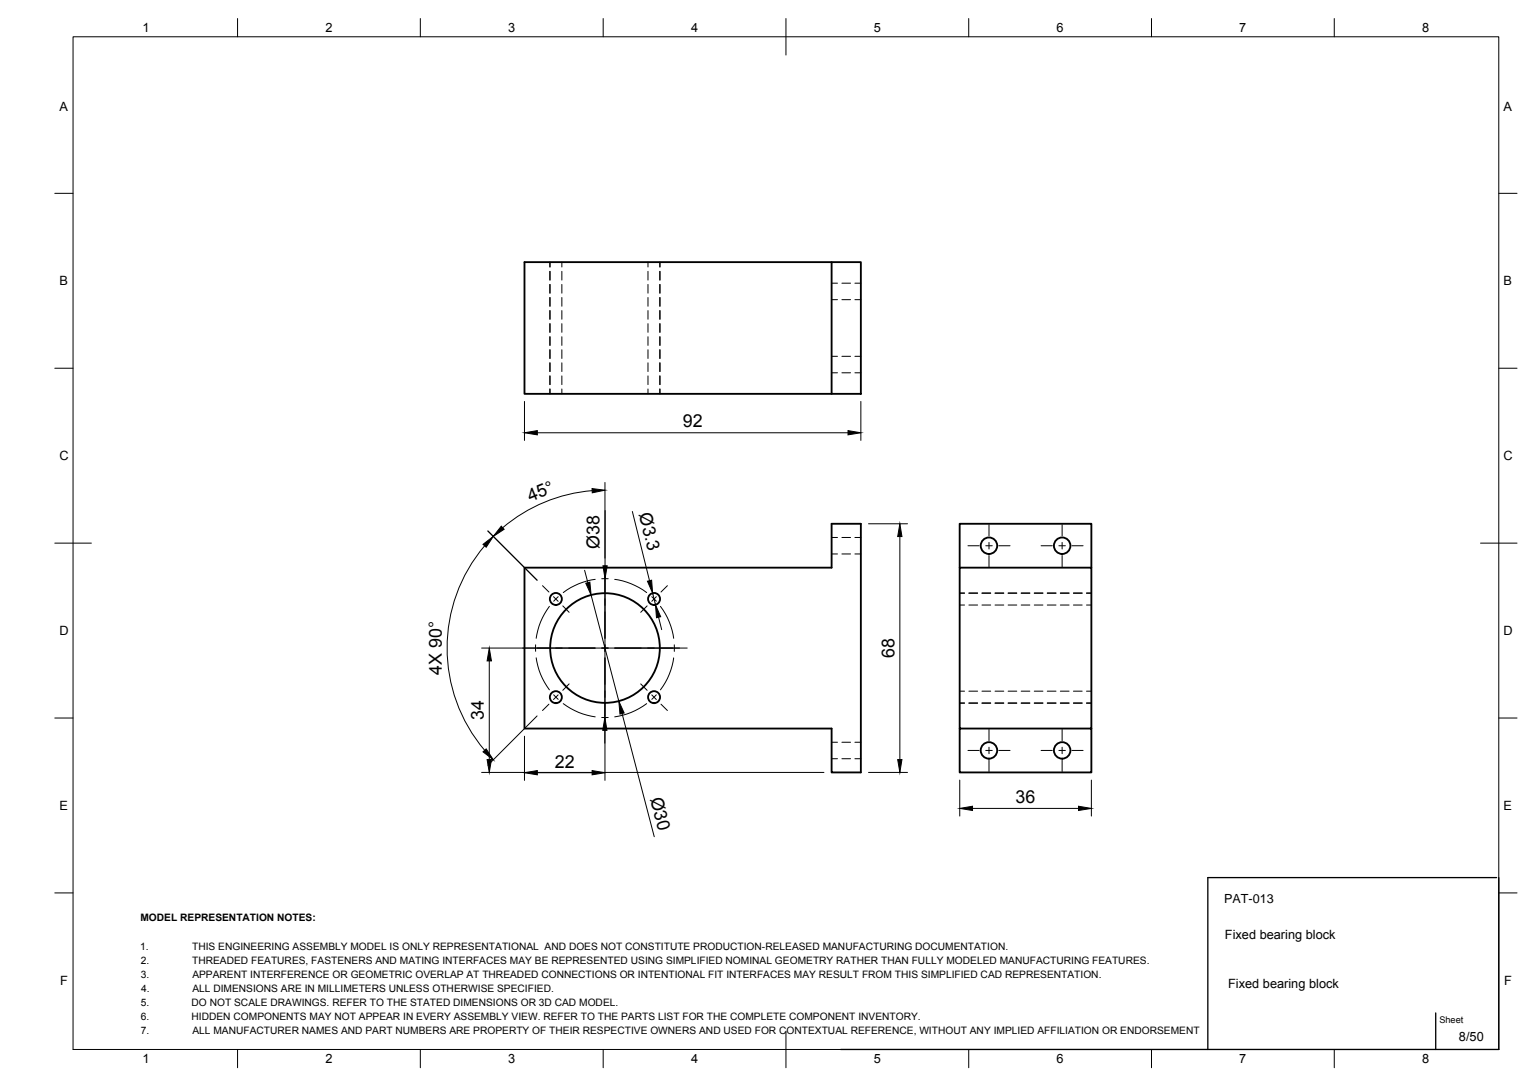
ISO-10303-21;
HEADER;
/* Generated by software containing ST-Developer
 * from STEP Tools, Inc. (www.steptools.com) 
 */

FILE_DESCRIPTION(
/* description */ ('Belt-driven linear axis on 2020 extrusion'),
/* implementation_level */ '2;1');

FILE_NAME(
/* name */ 'Fixed bearing block.step',
/* time_stamp */ '2026-10-28T03:26:09-07:00',
/* author */ (''),
/* organization */ (''),
/* preprocessor_version */ 'ST-DEVELOPER v20.2',
/* originating_system */ 'Autodesk Translation Framework v15.17.0.0',
/* authorisation */ '');

FILE_SCHEMA (('AUTOMOTIVE_DESIGN { 1 0 10303 214 3 1 1 }'));
ENDSEC;

DATA;
#10=MECHANICAL_DESIGN_GEOMETRIC_PRESENTATION_REPRESENTATION('',(#615),#20096);
#521=SHAPE_REPRESENTATION_RELATIONSHIP('SRR','None',#20317,#567);
#567=ADVANCED_BREP_SHAPE_REPRESENTATION('',(#671),#20048);
#615=STYLED_ITEM('',(#20650),#671);
#671=MANIFOLD_SOLID_BREP('Body1',#10928);
#742=FACE_BOUND('',#1972,.T.);
#743=FACE_BOUND('',#1973,.T.);
#744=FACE_BOUND('',#1975,.T.);
#745=FACE_BOUND('',#1976,.T.);
#746=FACE_BOUND('',#1980,.T.);
#747=FACE_BOUND('',#1981,.T.);
#748=FACE_BOUND('',#1982,.T.);
#749=FACE_BOUND('',#1983,.T.);
#750=FACE_BOUND('',#1984,.T.);
#751=FACE_BOUND('',#1987,.T.);
#752=FACE_BOUND('',#1988,.T.);
#753=FACE_BOUND('',#1989,.T.);
#754=FACE_BOUND('',#1990,.T.);
#755=FACE_BOUND('',#1991,.T.);
#756=FACE_BOUND('',#1995,.T.);
#757=FACE_BOUND('',#1996,.T.);
#758=FACE_BOUND('',#1997,.T.);
#759=FACE_BOUND('',#1998,.T.);
#935=PLANE('',#11629);
#936=PLANE('',#11630);
#937=PLANE('',#11631);
#938=PLANE('',#11632);
#939=PLANE('',#11633);
#940=PLANE('',#11634);
#941=PLANE('',#11635);
#942=PLANE('',#11636);
#943=PLANE('',#11637);
#944=PLANE('',#11638);
#1316=FACE_OUTER_BOUND('',#1962,.T.);
#1317=FACE_OUTER_BOUND('',#1963,.T.);
#1318=FACE_OUTER_BOUND('',#1964,.T.);
#1319=FACE_OUTER_BOUND('',#1965,.T.);
#1320=FACE_OUTER_BOUND('',#1966,.T.);
#1321=FACE_OUTER_BOUND('',#1967,.T.);
#1322=FACE_OUTER_BOUND('',#1968,.T.);
#1323=FACE_OUTER_BOUND('',#1969,.T.);
#1324=FACE_OUTER_BOUND('',#1970,.T.);
#1325=FACE_OUTER_BOUND('',#1971,.T.);
#1326=FACE_OUTER_BOUND('',#1974,.T.);
#1327=FACE_OUTER_BOUND('',#1977,.T.);
#1328=FACE_OUTER_BOUND('',#1978,.T.);
#1329=FACE_OUTER_BOUND('',#1979,.T.);
#1330=FACE_OUTER_BOUND('',#1985,.T.);
#1331=FACE_OUTER_BOUND('',#1986,.T.);
#1332=FACE_OUTER_BOUND('',#1992,.T.);
#1333=FACE_OUTER_BOUND('',#1993,.T.);
#1334=FACE_OUTER_BOUND('',#1994,.T.);
#1962=EDGE_LOOP('',(#7493,#7494,#7495,#7496));
#1963=EDGE_LOOP('',(#7497,#7498,#7499,#7500));
#1964=EDGE_LOOP('',(#7501,#7502,#7503,#7504));
#1965=EDGE_LOOP('',(#7505,#7506,#7507,#7508));
#1966=EDGE_LOOP('',(#7509,#7510,#7511,#7512));
#1967=EDGE_LOOP('',(#7513,#7514,#7515,#7516));
#1968=EDGE_LOOP('',(#7517,#7518,#7519,#7520));
#1969=EDGE_LOOP('',(#7521,#7522,#7523,#7524));
#1970=EDGE_LOOP('',(#7525,#7526,#7527,#7528));
#1971=EDGE_LOOP('',(#7529,#7530,#7531,#7532));
#1972=EDGE_LOOP('',(#7533));
#1973=EDGE_LOOP('',(#7534));
#1974=EDGE_LOOP('',(#7535,#7536,#7537,#7538));
#1975=EDGE_LOOP('',(#7539));
#1976=EDGE_LOOP('',(#7540));
#1977=EDGE_LOOP('',(#7541,#7542,#7543,#7544));
#1978=EDGE_LOOP('',(#7545,#7546,#7547,#7548));
#1979=EDGE_LOOP('',(#7549,#7550,#7551,#7552,#7553,#7554,#7555,#7556));
#1980=EDGE_LOOP('',(#7557));
#1981=EDGE_LOOP('',(#7558));
#1982=EDGE_LOOP('',(#7559));
#1983=EDGE_LOOP('',(#7560));
#1984=EDGE_LOOP('',(#7561));
#1985=EDGE_LOOP('',(#7562,#7563,#7564,#7565));
#1986=EDGE_LOOP('',(#7566,#7567,#7568,#7569,#7570,#7571,#7572,#7573));
#1987=EDGE_LOOP('',(#7574));
#1988=EDGE_LOOP('',(#7575));
#1989=EDGE_LOOP('',(#7576));
#1990=EDGE_LOOP('',(#7577));
#1991=EDGE_LOOP('',(#7578));
#1992=EDGE_LOOP('',(#7579,#7580,#7581,#7582));
#1993=EDGE_LOOP('',(#7583,#7584,#7585,#7586));
#1994=EDGE_LOOP('',(#7587,#7588,#7589,#7590));
#1995=EDGE_LOOP('',(#7591));
#1996=EDGE_LOOP('',(#7592));
#1997=EDGE_LOOP('',(#7593));
#1998=EDGE_LOOP('',(#7594));
#2745=LINE('',#16508,#3602);
#2746=LINE('',#16514,#3603);
#2747=LINE('',#16520,#3604);
#2748=LINE('',#16526,#3605);
#2749=LINE('',#16532,#3606);
#2750=LINE('',#16538,#3607);
#2751=LINE('',#16544,#3608);
#2752=LINE('',#16550,#3609);
#2753=LINE('',#16556,#3610);
#2754=LINE('',#16561,#3611);
#2755=LINE('',#16563,#3612);
#2756=LINE('',#16565,#3613);
#2757=LINE('',#16566,#3614);
#2758=LINE('',#16570,#3615);
#2759=LINE('',#16572,#3616);
#2760=LINE('',#16574,#3617);
#2761=LINE('',#16575,#3618);
#2762=LINE('',#16578,#3619);
#2763=LINE('',#16580,#3620);
#2764=LINE('',#16581,#3621);
#2765=LINE('',#16584,#3622);
#2766=LINE('',#16586,#3623);
#2767=LINE('',#16587,#3624);
#2768=LINE('',#16590,#3625);
#2769=LINE('',#16592,#3626);
#2770=LINE('',#16593,#3627);
#2771=LINE('',#16594,#3628);
#2772=LINE('',#16597,#3629);
#2773=LINE('',#16598,#3630);
#2774=LINE('',#16601,#3631);
#2775=LINE('',#16602,#3632);
#2776=LINE('',#16603,#3633);
#2777=LINE('',#16605,#3634);
#3602=VECTOR('',#13093,0.165);
#3603=VECTOR('',#13100,0.165);
#3604=VECTOR('',#13107,0.165);
#3605=VECTOR('',#13114,0.165);
#3606=VECTOR('',#13121,1.5);
#3607=VECTOR('',#13128,0.225);
#3608=VECTOR('',#13135,0.225);
#3609=VECTOR('',#13142,0.225);
#3610=VECTOR('',#13149,0.225);
#3611=VECTOR('',#13154,1.);
#3612=VECTOR('',#13155,1.);
#3613=VECTOR('',#13156,1.);
#3614=VECTOR('',#13157,1.);
#3615=VECTOR('',#13160,1.);
#3616=VECTOR('',#13161,1.);
#3617=VECTOR('',#13162,1.);
#3618=VECTOR('',#13163,1.);
#3619=VECTOR('',#13166,1.);
#3620=VECTOR('',#13167,1.);
#3621=VECTOR('',#13168,1.);
#3622=VECTOR('',#13171,1.);
#3623=VECTOR('',#13172,1.);
#3624=VECTOR('',#13173,1.);
#3625=VECTOR('',#13176,1.);
#3626=VECTOR('',#13177,1.);
#3627=VECTOR('',#13178,1.);
#3628=VECTOR('',#13179,1.);
#3629=VECTOR('',#13182,1.);
#3630=VECTOR('',#13183,1.);
#3631=VECTOR('',#13186,1.);
#3632=VECTOR('',#13187,1.);
#3633=VECTOR('',#13188,1.);
#3634=VECTOR('',#13191,1.);
#4419=CIRCLE('',#11603,0.165);
#4420=CIRCLE('',#11604,0.165);
#4421=CIRCLE('',#11606,0.165);
#4422=CIRCLE('',#11607,0.165);
#4423=CIRCLE('',#11609,0.165);
#4424=CIRCLE('',#11610,0.165);
#4425=CIRCLE('',#11612,0.165);
#4426=CIRCLE('',#11613,0.165);
#4427=CIRCLE('',#11615,1.5);
#4428=CIRCLE('',#11616,1.5);
#4429=CIRCLE('',#11618,0.225);
#4430=CIRCLE('',#11619,0.225);
#4431=CIRCLE('',#11621,0.225);
#4432=CIRCLE('',#11622,0.225);
#4433=CIRCLE('',#11624,0.225);
#4434=CIRCLE('',#11625,0.225);
#4435=CIRCLE('',#11627,0.225);
#4436=CIRCLE('',#11628,0.225);
#4972=VERTEX_POINT('',#16505);
#4973=VERTEX_POINT('',#16507);
#4974=VERTEX_POINT('',#16511);
#4975=VERTEX_POINT('',#16513);
#4976=VERTEX_POINT('',#16517);
#4977=VERTEX_POINT('',#16519);
#4978=VERTEX_POINT('',#16523);
#4979=VERTEX_POINT('',#16525);
#4980=VERTEX_POINT('',#16529);
#4981=VERTEX_POINT('',#16531);
#4982=VERTEX_POINT('',#16535);
#4983=VERTEX_POINT('',#16537);
#4984=VERTEX_POINT('',#16541);
#4985=VERTEX_POINT('',#16543);
#4986=VERTEX_POINT('',#16547);
#4987=VERTEX_POINT('',#16549);
#4988=VERTEX_POINT('',#16553);
#4989=VERTEX_POINT('',#16555);
#4990=VERTEX_POINT('',#16559);
#4991=VERTEX_POINT('',#16560);
#4992=VERTEX_POINT('',#16562);
#4993=VERTEX_POINT('',#16564);
#4994=VERTEX_POINT('',#16568);
#4995=VERTEX_POINT('',#16569);
#4996=VERTEX_POINT('',#16571);
#4997=VERTEX_POINT('',#16573);
#4998=VERTEX_POINT('',#16577);
#4999=VERTEX_POINT('',#16579);
#5000=VERTEX_POINT('',#16583);
#5001=VERTEX_POINT('',#16585);
#5002=VERTEX_POINT('',#16589);
#5003=VERTEX_POINT('',#16591);
#5004=VERTEX_POINT('',#16596);
#5005=VERTEX_POINT('',#16600);
#5961=EDGE_CURVE('',#4972,#4972,#4419,.T.);
#5962=EDGE_CURVE('',#4972,#4973,#2745,.T.);
#5963=EDGE_CURVE('',#4973,#4973,#4420,.T.);
#5964=EDGE_CURVE('',#4974,#4974,#4421,.T.);
#5965=EDGE_CURVE('',#4974,#4975,#2746,.T.);
#5966=EDGE_CURVE('',#4975,#4975,#4422,.T.);
#5967=EDGE_CURVE('',#4976,#4976,#4423,.T.);
#5968=EDGE_CURVE('',#4976,#4977,#2747,.T.);
#5969=EDGE_CURVE('',#4977,#4977,#4424,.T.);
#5970=EDGE_CURVE('',#4978,#4978,#4425,.T.);
#5971=EDGE_CURVE('',#4978,#4979,#2748,.T.);
#5972=EDGE_CURVE('',#4979,#4979,#4426,.T.);
#5973=EDGE_CURVE('',#4980,#4980,#4427,.T.);
#5974=EDGE_CURVE('',#4980,#4981,#2749,.T.);
#5975=EDGE_CURVE('',#4981,#4981,#4428,.T.);
#5976=EDGE_CURVE('',#4982,#4982,#4429,.T.);
#5977=EDGE_CURVE('',#4982,#4983,#2750,.T.);
#5978=EDGE_CURVE('',#4983,#4983,#4430,.T.);
#5979=EDGE_CURVE('',#4984,#4984,#4431,.T.);
#5980=EDGE_CURVE('',#4984,#4985,#2751,.T.);
#5981=EDGE_CURVE('',#4985,#4985,#4432,.T.);
#5982=EDGE_CURVE('',#4986,#4986,#4433,.T.);
#5983=EDGE_CURVE('',#4986,#4987,#2752,.T.);
#5984=EDGE_CURVE('',#4987,#4987,#4434,.T.);
#5985=EDGE_CURVE('',#4988,#4988,#4435,.T.);
#5986=EDGE_CURVE('',#4988,#4989,#2753,.T.);
#5987=EDGE_CURVE('',#4989,#4989,#4436,.T.);
#5988=EDGE_CURVE('',#4990,#4991,#2754,.T.);
#5989=EDGE_CURVE('',#4992,#4990,#2755,.T.);
#5990=EDGE_CURVE('',#4992,#4993,#2756,.T.);
#5991=EDGE_CURVE('',#4991,#4993,#2757,.T.);
#5992=EDGE_CURVE('',#4994,#4995,#2758,.T.);
#5993=EDGE_CURVE('',#4996,#4994,#2759,.T.);
#5994=EDGE_CURVE('',#4997,#4996,#2760,.T.);
#5995=EDGE_CURVE('',#4995,#4997,#2761,.T.);
#5996=EDGE_CURVE('',#4997,#4998,#2762,.T.);
#5997=EDGE_CURVE('',#4999,#4996,#2763,.T.);
#5998=EDGE_CURVE('',#4998,#4999,#2764,.T.);
#5999=EDGE_CURVE('',#5000,#4992,#2765,.T.);
#6000=EDGE_CURVE('',#5000,#5001,#2766,.T.);
#6001=EDGE_CURVE('',#4993,#5001,#2767,.T.);
#6002=EDGE_CURVE('',#4990,#5002,#2768,.T.);
#6003=EDGE_CURVE('',#5003,#5002,#2769,.T.);
#6004=EDGE_CURVE('',#4995,#5003,#2770,.T.);
#6005=EDGE_CURVE('',#4998,#5000,#2771,.T.);
#6006=EDGE_CURVE('',#4991,#5004,#2772,.T.);
#6007=EDGE_CURVE('',#5002,#5004,#2773,.T.);
#6008=EDGE_CURVE('',#4994,#5005,#2774,.T.);
#6009=EDGE_CURVE('',#5004,#5005,#2775,.T.);
#6010=EDGE_CURVE('',#5001,#4999,#2776,.T.);
#6011=EDGE_CURVE('',#5005,#5003,#2777,.T.);
#7493=ORIENTED_EDGE('',*,*,#5961,.F.);
#7494=ORIENTED_EDGE('',*,*,#5962,.T.);
#7495=ORIENTED_EDGE('',*,*,#5963,.F.);
#7496=ORIENTED_EDGE('',*,*,#5962,.F.);
#7497=ORIENTED_EDGE('',*,*,#5964,.F.);
#7498=ORIENTED_EDGE('',*,*,#5965,.T.);
#7499=ORIENTED_EDGE('',*,*,#5966,.F.);
#7500=ORIENTED_EDGE('',*,*,#5965,.F.);
#7501=ORIENTED_EDGE('',*,*,#5967,.F.);
#7502=ORIENTED_EDGE('',*,*,#5968,.T.);
#7503=ORIENTED_EDGE('',*,*,#5969,.F.);
#7504=ORIENTED_EDGE('',*,*,#5968,.F.);
#7505=ORIENTED_EDGE('',*,*,#5970,.F.);
#7506=ORIENTED_EDGE('',*,*,#5971,.T.);
#7507=ORIENTED_EDGE('',*,*,#5972,.F.);
#7508=ORIENTED_EDGE('',*,*,#5971,.F.);
#7509=ORIENTED_EDGE('',*,*,#5973,.F.);
#7510=ORIENTED_EDGE('',*,*,#5974,.T.);
#7511=ORIENTED_EDGE('',*,*,#5975,.F.);
#7512=ORIENTED_EDGE('',*,*,#5974,.F.);
#7513=ORIENTED_EDGE('',*,*,#5976,.F.);
#7514=ORIENTED_EDGE('',*,*,#5977,.T.);
#7515=ORIENTED_EDGE('',*,*,#5978,.F.);
#7516=ORIENTED_EDGE('',*,*,#5977,.F.);
#7517=ORIENTED_EDGE('',*,*,#5979,.F.);
#7518=ORIENTED_EDGE('',*,*,#5980,.T.);
#7519=ORIENTED_EDGE('',*,*,#5981,.F.);
#7520=ORIENTED_EDGE('',*,*,#5980,.F.);
#7521=ORIENTED_EDGE('',*,*,#5982,.F.);
#7522=ORIENTED_EDGE('',*,*,#5983,.T.);
#7523=ORIENTED_EDGE('',*,*,#5984,.F.);
#7524=ORIENTED_EDGE('',*,*,#5983,.F.);
#7525=ORIENTED_EDGE('',*,*,#5985,.F.);
#7526=ORIENTED_EDGE('',*,*,#5986,.T.);
#7527=ORIENTED_EDGE('',*,*,#5987,.F.);
#7528=ORIENTED_EDGE('',*,*,#5986,.F.);
#7529=ORIENTED_EDGE('',*,*,#5988,.F.);
#7530=ORIENTED_EDGE('',*,*,#5989,.F.);
#7531=ORIENTED_EDGE('',*,*,#5990,.T.);
#7532=ORIENTED_EDGE('',*,*,#5991,.F.);
#7533=ORIENTED_EDGE('',*,*,#5978,.T.);
#7534=ORIENTED_EDGE('',*,*,#5987,.T.);
#7535=ORIENTED_EDGE('',*,*,#5992,.F.);
#7536=ORIENTED_EDGE('',*,*,#5993,.F.);
#7537=ORIENTED_EDGE('',*,*,#5994,.F.);
#7538=ORIENTED_EDGE('',*,*,#5995,.F.);
#7539=ORIENTED_EDGE('',*,*,#5981,.T.);
#7540=ORIENTED_EDGE('',*,*,#5984,.T.);
#7541=ORIENTED_EDGE('',*,*,#5996,.F.);
#7542=ORIENTED_EDGE('',*,*,#5994,.T.);
#7543=ORIENTED_EDGE('',*,*,#5997,.F.);
#7544=ORIENTED_EDGE('',*,*,#5998,.F.);
#7545=ORIENTED_EDGE('',*,*,#5999,.F.);
#7546=ORIENTED_EDGE('',*,*,#6000,.T.);
#7547=ORIENTED_EDGE('',*,*,#6001,.F.);
#7548=ORIENTED_EDGE('',*,*,#5990,.F.);
#7549=ORIENTED_EDGE('',*,*,#6002,.T.);
#7550=ORIENTED_EDGE('',*,*,#6003,.F.);
#7551=ORIENTED_EDGE('',*,*,#6004,.F.);
#7552=ORIENTED_EDGE('',*,*,#5995,.T.);
#7553=ORIENTED_EDGE('',*,*,#5996,.T.);
#7554=ORIENTED_EDGE('',*,*,#6005,.T.);
#7555=ORIENTED_EDGE('',*,*,#5999,.T.);
#7556=ORIENTED_EDGE('',*,*,#5989,.T.);
#7557=ORIENTED_EDGE('',*,*,#5973,.T.);
#7558=ORIENTED_EDGE('',*,*,#5970,.T.);
#7559=ORIENTED_EDGE('',*,*,#5967,.T.);
#7560=ORIENTED_EDGE('',*,*,#5964,.T.);
#7561=ORIENTED_EDGE('',*,*,#5961,.T.);
#7562=ORIENTED_EDGE('',*,*,#5988,.T.);
#7563=ORIENTED_EDGE('',*,*,#6006,.T.);
#7564=ORIENTED_EDGE('',*,*,#6007,.F.);
#7565=ORIENTED_EDGE('',*,*,#6002,.F.);
#7566=ORIENTED_EDGE('',*,*,#6008,.T.);
#7567=ORIENTED_EDGE('',*,*,#6009,.F.);
#7568=ORIENTED_EDGE('',*,*,#6006,.F.);
#7569=ORIENTED_EDGE('',*,*,#5991,.T.);
#7570=ORIENTED_EDGE('',*,*,#6001,.T.);
#7571=ORIENTED_EDGE('',*,*,#6010,.T.);
#7572=ORIENTED_EDGE('',*,*,#5997,.T.);
#7573=ORIENTED_EDGE('',*,*,#5993,.T.);
#7574=ORIENTED_EDGE('',*,*,#5975,.T.);
#7575=ORIENTED_EDGE('',*,*,#5972,.T.);
#7576=ORIENTED_EDGE('',*,*,#5969,.T.);
#7577=ORIENTED_EDGE('',*,*,#5966,.T.);
#7578=ORIENTED_EDGE('',*,*,#5963,.T.);
#7579=ORIENTED_EDGE('',*,*,#5992,.T.);
#7580=ORIENTED_EDGE('',*,*,#6004,.T.);
#7581=ORIENTED_EDGE('',*,*,#6011,.F.);
#7582=ORIENTED_EDGE('',*,*,#6008,.F.);
#7583=ORIENTED_EDGE('',*,*,#6011,.T.);
#7584=ORIENTED_EDGE('',*,*,#6003,.T.);
#7585=ORIENTED_EDGE('',*,*,#6007,.T.);
#7586=ORIENTED_EDGE('',*,*,#6009,.T.);
#7587=ORIENTED_EDGE('',*,*,#6010,.F.);
#7588=ORIENTED_EDGE('',*,*,#6000,.F.);
#7589=ORIENTED_EDGE('',*,*,#6005,.F.);
#7590=ORIENTED_EDGE('',*,*,#5998,.T.);
#7591=ORIENTED_EDGE('',*,*,#5976,.T.);
#7592=ORIENTED_EDGE('',*,*,#5979,.T.);
#7593=ORIENTED_EDGE('',*,*,#5982,.T.);
#7594=ORIENTED_EDGE('',*,*,#5985,.T.);
#10097=CYLINDRICAL_SURFACE('',#11602,0.165);
#10098=CYLINDRICAL_SURFACE('',#11605,0.165);
#10099=CYLINDRICAL_SURFACE('',#11608,0.165);
#10100=CYLINDRICAL_SURFACE('',#11611,0.165);
#10101=CYLINDRICAL_SURFACE('',#11614,1.5);
#10102=CYLINDRICAL_SURFACE('',#11617,0.225);
#10103=CYLINDRICAL_SURFACE('',#11620,0.225);
#10104=CYLINDRICAL_SURFACE('',#11623,0.225);
#10105=CYLINDRICAL_SURFACE('',#11626,0.225);
#10367=ADVANCED_FACE('',(#1316),#10097,.F.);
#10368=ADVANCED_FACE('',(#1317),#10098,.F.);
#10369=ADVANCED_FACE('',(#1318),#10099,.F.);
#10370=ADVANCED_FACE('',(#1319),#10100,.F.);
#10371=ADVANCED_FACE('',(#1320),#10101,.F.);
#10372=ADVANCED_FACE('',(#1321),#10102,.F.);
#10373=ADVANCED_FACE('',(#1322),#10103,.F.);
#10374=ADVANCED_FACE('',(#1323),#10104,.F.);
#10375=ADVANCED_FACE('',(#1324),#10105,.F.);
#10376=ADVANCED_FACE('',(#1325,#742,#743),#935,.T.);
#10377=ADVANCED_FACE('',(#1326,#744,#745),#936,.T.);
#10378=ADVANCED_FACE('',(#1327),#937,.T.);
#10379=ADVANCED_FACE('',(#1328),#938,.T.);
#10380=ADVANCED_FACE('',(#1329,#746,#747,#748,#749,#750),#939,.T.);
#10381=ADVANCED_FACE('',(#1330),#940,.T.);
#10382=ADVANCED_FACE('',(#1331,#751,#752,#753,#754,#755),#941,.T.);
#10383=ADVANCED_FACE('',(#1332),#942,.T.);
#10384=ADVANCED_FACE('',(#1333),#943,.T.);
#10385=ADVANCED_FACE('',(#1334,#756,#757,#758,#759),#944,.F.);
#10928=CLOSED_SHELL('',(#10367,#10368,#10369,#10370,#10371,#10372,#10373,
#10374,#10375,#10376,#10377,#10378,#10379,#10380,#10381,#10382,#10383,#10384,
#10385));
#11601=AXIS2_PLACEMENT_3D('',#16503,#13087,#13088);
#11602=AXIS2_PLACEMENT_3D('',#16504,#13089,#13090);
#11603=AXIS2_PLACEMENT_3D('',#16506,#13091,#13092);
#11604=AXIS2_PLACEMENT_3D('',#16509,#13094,#13095);
#11605=AXIS2_PLACEMENT_3D('',#16510,#13096,#13097);
#11606=AXIS2_PLACEMENT_3D('',#16512,#13098,#13099);
#11607=AXIS2_PLACEMENT_3D('',#16515,#13101,#13102);
#11608=AXIS2_PLACEMENT_3D('',#16516,#13103,#13104);
#11609=AXIS2_PLACEMENT_3D('',#16518,#13105,#13106);
#11610=AXIS2_PLACEMENT_3D('',#16521,#13108,#13109);
#11611=AXIS2_PLACEMENT_3D('',#16522,#13110,#13111);
#11612=AXIS2_PLACEMENT_3D('',#16524,#13112,#13113);
#11613=AXIS2_PLACEMENT_3D('',#16527,#13115,#13116);
#11614=AXIS2_PLACEMENT_3D('',#16528,#13117,#13118);
#11615=AXIS2_PLACEMENT_3D('',#16530,#13119,#13120);
#11616=AXIS2_PLACEMENT_3D('',#16533,#13122,#13123);
#11617=AXIS2_PLACEMENT_3D('',#16534,#13124,#13125);
#11618=AXIS2_PLACEMENT_3D('',#16536,#13126,#13127);
#11619=AXIS2_PLACEMENT_3D('',#16539,#13129,#13130);
#11620=AXIS2_PLACEMENT_3D('',#16540,#13131,#13132);
#11621=AXIS2_PLACEMENT_3D('',#16542,#13133,#13134);
#11622=AXIS2_PLACEMENT_3D('',#16545,#13136,#13137);
#11623=AXIS2_PLACEMENT_3D('',#16546,#13138,#13139);
#11624=AXIS2_PLACEMENT_3D('',#16548,#13140,#13141);
#11625=AXIS2_PLACEMENT_3D('',#16551,#13143,#13144);
#11626=AXIS2_PLACEMENT_3D('',#16552,#13145,#13146);
#11627=AXIS2_PLACEMENT_3D('',#16554,#13147,#13148);
#11628=AXIS2_PLACEMENT_3D('',#16557,#13150,#13151);
#11629=AXIS2_PLACEMENT_3D('',#16558,#13152,#13153);
#11630=AXIS2_PLACEMENT_3D('',#16567,#13158,#13159);
#11631=AXIS2_PLACEMENT_3D('',#16576,#13164,#13165);
#11632=AXIS2_PLACEMENT_3D('',#16582,#13169,#13170);
#11633=AXIS2_PLACEMENT_3D('',#16588,#13174,#13175);
#11634=AXIS2_PLACEMENT_3D('',#16595,#13180,#13181);
#11635=AXIS2_PLACEMENT_3D('',#16599,#13184,#13185);
#11636=AXIS2_PLACEMENT_3D('',#16604,#13189,#13190);
#11637=AXIS2_PLACEMENT_3D('',#16606,#13192,#13193);
#11638=AXIS2_PLACEMENT_3D('',#16607,#13194,#13195);
#13087=DIRECTION('axis',(0.,0.,1.));
#13088=DIRECTION('refdir',(1.,0.,0.));
#13089=DIRECTION('center_axis',(0.,1.,0.));
#13090=DIRECTION('ref_axis',(1.,0.,0.));
#13091=DIRECTION('center_axis',(0.,1.,0.));
#13092=DIRECTION('ref_axis',(1.,0.,0.));
#13093=DIRECTION('',(0.,1.,0.));
#13094=DIRECTION('center_axis',(0.,-1.,0.));
#13095=DIRECTION('ref_axis',(1.,0.,0.));
#13096=DIRECTION('center_axis',(0.,1.,0.));
#13097=DIRECTION('ref_axis',(1.,0.,0.));
#13098=DIRECTION('center_axis',(0.,1.,0.));
#13099=DIRECTION('ref_axis',(1.,0.,0.));
#13100=DIRECTION('',(0.,1.,0.));
#13101=DIRECTION('center_axis',(0.,-1.,0.));
#13102=DIRECTION('ref_axis',(1.,0.,0.));
#13103=DIRECTION('center_axis',(0.,1.,0.));
#13104=DIRECTION('ref_axis',(1.,0.,0.));
#13105=DIRECTION('center_axis',(0.,1.,0.));
#13106=DIRECTION('ref_axis',(1.,0.,0.));
#13107=DIRECTION('',(0.,1.,0.));
#13108=DIRECTION('center_axis',(0.,-1.,0.));
#13109=DIRECTION('ref_axis',(1.,0.,0.));
#13110=DIRECTION('center_axis',(0.,1.,0.));
#13111=DIRECTION('ref_axis',(1.,0.,0.));
#13112=DIRECTION('center_axis',(0.,1.,0.));
#13113=DIRECTION('ref_axis',(1.,0.,0.));
#13114=DIRECTION('',(0.,1.,0.));
#13115=DIRECTION('center_axis',(0.,-1.,0.));
#13116=DIRECTION('ref_axis',(1.,0.,0.));
#13117=DIRECTION('center_axis',(0.,1.,0.));
#13118=DIRECTION('ref_axis',(1.,0.,0.));
#13119=DIRECTION('center_axis',(0.,1.,0.));
#13120=DIRECTION('ref_axis',(1.,0.,0.));
#13121=DIRECTION('',(0.,1.,0.));
#13122=DIRECTION('center_axis',(0.,-1.,0.));
#13123=DIRECTION('ref_axis',(1.,0.,0.));
#13124=DIRECTION('center_axis',(0.,0.,1.));
#13125=DIRECTION('ref_axis',(1.,0.,0.));
#13126=DIRECTION('center_axis',(0.,0.,1.));
#13127=DIRECTION('ref_axis',(1.,0.,0.));
#13128=DIRECTION('',(0.,0.,1.));
#13129=DIRECTION('center_axis',(0.,0.,-1.));
#13130=DIRECTION('ref_axis',(1.,0.,0.));
#13131=DIRECTION('center_axis',(0.,0.,1.));
#13132=DIRECTION('ref_axis',(1.,0.,0.));
#13133=DIRECTION('center_axis',(0.,0.,1.));
#13134=DIRECTION('ref_axis',(1.,0.,0.));
#13135=DIRECTION('',(0.,0.,1.));
#13136=DIRECTION('center_axis',(0.,0.,-1.));
#13137=DIRECTION('ref_axis',(1.,0.,0.));
#13138=DIRECTION('center_axis',(0.,0.,1.));
#13139=DIRECTION('ref_axis',(1.,0.,0.));
#13140=DIRECTION('center_axis',(0.,0.,1.));
#13141=DIRECTION('ref_axis',(1.,0.,0.));
#13142=DIRECTION('',(0.,0.,1.));
#13143=DIRECTION('center_axis',(0.,0.,-1.));
#13144=DIRECTION('ref_axis',(1.,0.,0.));
#13145=DIRECTION('center_axis',(0.,0.,1.));
#13146=DIRECTION('ref_axis',(1.,0.,0.));
#13147=DIRECTION('center_axis',(0.,0.,1.));
#13148=DIRECTION('ref_axis',(1.,0.,0.));
#13149=DIRECTION('',(0.,0.,1.));
#13150=DIRECTION('center_axis',(0.,0.,-1.));
#13151=DIRECTION('ref_axis',(1.,0.,0.));
#13152=DIRECTION('center_axis',(0.,0.,1.));
#13153=DIRECTION('ref_axis',(1.,0.,0.));
#13154=DIRECTION('',(0.,1.,0.));
#13155=DIRECTION('',(-1.,0.,0.));
#13156=DIRECTION('',(0.,1.,0.));
#13157=DIRECTION('',(1.,0.,0.));
#13158=DIRECTION('center_axis',(0.,0.,1.));
#13159=DIRECTION('ref_axis',(1.,0.,0.));
#13160=DIRECTION('',(0.,-1.,0.));
#13161=DIRECTION('',(1.,0.,0.));
#13162=DIRECTION('',(0.,1.,0.));
#13163=DIRECTION('',(-1.,0.,0.));
#13164=DIRECTION('center_axis',(-1.,0.,0.));
#13165=DIRECTION('ref_axis',(0.,0.,1.));
#13166=DIRECTION('',(0.,0.,-1.));
#13167=DIRECTION('',(0.,0.,1.));
#13168=DIRECTION('',(0.,1.,0.));
#13169=DIRECTION('center_axis',(1.,0.,0.));
#13170=DIRECTION('ref_axis',(0.,0.,-1.));
#13171=DIRECTION('',(0.,0.,1.));
#13172=DIRECTION('',(0.,1.,0.));
#13173=DIRECTION('',(0.,0.,-1.));
#13174=DIRECTION('center_axis',(0.,-1.,0.));
#13175=DIRECTION('ref_axis',(1.,0.,0.));
#13176=DIRECTION('',(0.,0.,1.));
#13177=DIRECTION('',(1.,0.,0.));
#13178=DIRECTION('',(0.,0.,1.));
#13179=DIRECTION('',(1.,0.,0.));
#13180=DIRECTION('center_axis',(1.,0.,0.));
#13181=DIRECTION('ref_axis',(0.,1.,0.));
#13182=DIRECTION('',(0.,0.,1.));
#13183=DIRECTION('',(0.,1.,0.));
#13184=DIRECTION('center_axis',(0.,1.,0.));
#13185=DIRECTION('ref_axis',(-1.,0.,0.));
#13186=DIRECTION('',(0.,0.,1.));
#13187=DIRECTION('',(-1.,0.,0.));
#13188=DIRECTION('',(-1.,0.,0.));
#13189=DIRECTION('center_axis',(-1.,0.,0.));
#13190=DIRECTION('ref_axis',(0.,-1.,0.));
#13191=DIRECTION('',(0.,-1.,0.));
#13192=DIRECTION('center_axis',(0.,0.,1.));
#13193=DIRECTION('ref_axis',(1.,0.,0.));
#13194=DIRECTION('center_axis',(0.,0.,1.));
#13195=DIRECTION('ref_axis',(1.,0.,0.));
#16503=CARTESIAN_POINT('',(0.,0.,0.));
#16504=CARTESIAN_POINT('Origin',(-1.34350288425444,-1.9,5.65649711574556));
#16505=CARTESIAN_POINT('',(-1.50850288425444,-1.8,5.65649711574556));
#16506=CARTESIAN_POINT('Origin',(-1.34350288425444,-1.8,5.65649711574556));
#16507=CARTESIAN_POINT('',(-1.50850288425444,1.8,5.65649711574556));
#16508=CARTESIAN_POINT('',(-1.50850288425444,-1.9,5.65649711574556));
#16509=CARTESIAN_POINT('Origin',(-1.34350288425444,1.8,5.65649711574556));
#16510=CARTESIAN_POINT('Origin',(-1.34350288425444,-1.9,8.34350288425444));
#16511=CARTESIAN_POINT('',(-1.50850288425444,-1.8,8.34350288425444));
#16512=CARTESIAN_POINT('Origin',(-1.34350288425444,-1.8,8.34350288425444));
#16513=CARTESIAN_POINT('',(-1.50850288425444,1.8,8.34350288425444));
#16514=CARTESIAN_POINT('',(-1.50850288425444,-1.9,8.34350288425444));
#16515=CARTESIAN_POINT('Origin',(-1.34350288425444,1.8,8.34350288425444));
#16516=CARTESIAN_POINT('Origin',(1.34350288425444,-1.9,8.34350288425444));
#16517=CARTESIAN_POINT('',(1.17850288425444,-1.8,8.34350288425444));
#16518=CARTESIAN_POINT('Origin',(1.34350288425444,-1.8,8.34350288425444));
#16519=CARTESIAN_POINT('',(1.17850288425444,1.8,8.34350288425444));
#16520=CARTESIAN_POINT('',(1.17850288425444,-1.9,8.34350288425444));
#16521=CARTESIAN_POINT('Origin',(1.34350288425444,1.8,8.34350288425444));
#16522=CARTESIAN_POINT('Origin',(1.34350288425444,-1.9,5.65649711574556));
#16523=CARTESIAN_POINT('',(1.17850288425444,-1.8,5.65649711574556));
#16524=CARTESIAN_POINT('Origin',(1.34350288425444,-1.8,5.65649711574556));
#16525=CARTESIAN_POINT('',(1.17850288425444,1.8,5.65649711574556));
#16526=CARTESIAN_POINT('',(1.17850288425444,-1.9,5.65649711574556));
#16527=CARTESIAN_POINT('Origin',(1.34350288425444,1.8,5.65649711574556));
#16528=CARTESIAN_POINT('Origin',(0.,-1.9,7.));
#16529=CARTESIAN_POINT('',(-1.5,-1.8,7.));
#16530=CARTESIAN_POINT('Origin',(0.,-1.8,7.));
#16531=CARTESIAN_POINT('',(-1.5,1.8,7.));
#16532=CARTESIAN_POINT('',(-1.5,-1.9,7.));
#16533=CARTESIAN_POINT('Origin',(0.,1.8,7.));
#16534=CARTESIAN_POINT('Origin',(2.8,-1.,-0.1));
#16535=CARTESIAN_POINT('',(2.575,-1.,0.));
#16536=CARTESIAN_POINT('Origin',(2.8,-1.,0.));
#16537=CARTESIAN_POINT('',(2.575,-1.,0.8));
#16538=CARTESIAN_POINT('',(2.575,-1.,-0.1));
#16539=CARTESIAN_POINT('Origin',(2.8,-1.,0.8));
#16540=CARTESIAN_POINT('Origin',(-2.8,1.,-0.1));
#16541=CARTESIAN_POINT('',(-3.025,1.,0.));
#16542=CARTESIAN_POINT('Origin',(-2.8,1.,0.));
#16543=CARTESIAN_POINT('',(-3.025,1.,0.8));
#16544=CARTESIAN_POINT('',(-3.025,1.,-0.1));
#16545=CARTESIAN_POINT('Origin',(-2.8,1.,0.8));
#16546=CARTESIAN_POINT('Origin',(-2.8,-1.,-0.1));
#16547=CARTESIAN_POINT('',(-3.025,-1.,0.));
#16548=CARTESIAN_POINT('Origin',(-2.8,-1.,0.));
#16549=CARTESIAN_POINT('',(-3.025,-1.,0.8));
#16550=CARTESIAN_POINT('',(-3.025,-1.,-0.1));
#16551=CARTESIAN_POINT('Origin',(-2.8,-1.,0.8));
#16552=CARTESIAN_POINT('Origin',(2.8,1.,-0.1));
#16553=CARTESIAN_POINT('',(2.575,1.,0.));
#16554=CARTESIAN_POINT('Origin',(2.8,1.,0.));
#16555=CARTESIAN_POINT('',(2.575,1.,0.8));
#16556=CARTESIAN_POINT('',(2.575,1.,-0.1));
#16557=CARTESIAN_POINT('Origin',(2.8,1.,0.8));
#16558=CARTESIAN_POINT('Origin',(-3.4,-1.8,0.8));
#16559=CARTESIAN_POINT('',(2.2,-1.8,0.8));
#16560=CARTESIAN_POINT('',(2.2,1.8,0.8));
#16561=CARTESIAN_POINT('',(2.2,-1.8,0.8));
#16562=CARTESIAN_POINT('',(3.4,-1.8,0.8));
#16563=CARTESIAN_POINT('',(3.4,-1.8,0.8));
#16564=CARTESIAN_POINT('',(3.4,1.8,0.8));
#16565=CARTESIAN_POINT('',(3.4,-1.8,0.8));
#16566=CARTESIAN_POINT('',(3.4,1.8,0.8));
#16567=CARTESIAN_POINT('Origin',(-3.4,-1.8,0.8));
#16568=CARTESIAN_POINT('',(-2.2,1.8,0.8));
#16569=CARTESIAN_POINT('',(-2.2,-1.8,0.8));
#16570=CARTESIAN_POINT('',(-2.2,0.,0.8));
#16571=CARTESIAN_POINT('',(-3.4,1.8,0.8));
#16572=CARTESIAN_POINT('',(3.4,1.8,0.8));
#16573=CARTESIAN_POINT('',(-3.4,-1.8,0.8));
#16574=CARTESIAN_POINT('',(-3.4,-1.8,0.8));
#16575=CARTESIAN_POINT('',(3.4,-1.8,0.8));
#16576=CARTESIAN_POINT('Origin',(-3.4,-1.8,0.));
#16577=CARTESIAN_POINT('',(-3.4,-1.8,0.));
#16578=CARTESIAN_POINT('',(-3.4,-1.8,0.8));
#16579=CARTESIAN_POINT('',(-3.4,1.8,0.));
#16580=CARTESIAN_POINT('',(-3.4,1.8,0.8));
#16581=CARTESIAN_POINT('',(-3.4,-1.8,0.));
#16582=CARTESIAN_POINT('Origin',(3.4,-1.8,0.8));
#16583=CARTESIAN_POINT('',(3.4,-1.8,0.));
#16584=CARTESIAN_POINT('',(3.4,-1.8,0.));
#16585=CARTESIAN_POINT('',(3.4,1.8,0.));
#16586=CARTESIAN_POINT('',(3.4,-1.8,0.));
#16587=CARTESIAN_POINT('',(3.4,1.8,0.));
#16588=CARTESIAN_POINT('Origin',(-2.2,-1.8,0.));
#16589=CARTESIAN_POINT('',(2.2,-1.8,9.2));
#16590=CARTESIAN_POINT('',(2.2,-1.8,0.));
#16591=CARTESIAN_POINT('',(-2.2,-1.8,9.2));
#16592=CARTESIAN_POINT('',(-2.2,-1.8,9.2));
#16593=CARTESIAN_POINT('',(-2.2,-1.8,0.));
#16594=CARTESIAN_POINT('',(-3.4,-1.8,0.));
#16595=CARTESIAN_POINT('Origin',(2.2,-1.8,0.));
#16596=CARTESIAN_POINT('',(2.2,1.8,9.2));
#16597=CARTESIAN_POINT('',(2.2,1.8,0.));
#16598=CARTESIAN_POINT('',(2.2,-1.8,9.2));
#16599=CARTESIAN_POINT('Origin',(2.2,1.8,0.));
#16600=CARTESIAN_POINT('',(-2.2,1.8,9.2));
#16601=CARTESIAN_POINT('',(-2.2,1.8,0.));
#16602=CARTESIAN_POINT('',(2.2,1.8,9.2));
#16603=CARTESIAN_POINT('',(-3.4,1.8,0.));
#16604=CARTESIAN_POINT('Origin',(-2.2,1.8,0.));
#16605=CARTESIAN_POINT('',(-2.2,1.8,9.2));
#16606=CARTESIAN_POINT('Origin',(0.,0.,9.2));
#16607=CARTESIAN_POINT('Origin',(0.,0.,0.));
#19994=UNCERTAINTY_MEASURE_WITH_UNIT(LENGTH_MEASURE(0.001),#20097,
'DISTANCE_ACCURACY_VALUE',
'Maximum model space distance between geometric entities at asserted c
onnectivities');
#20042=UNCERTAINTY_MEASURE_WITH_UNIT(LENGTH_MEASURE(0.001),#20097,
'DISTANCE_ACCURACY_VALUE',
'Maximum model space distance between geometric entities at asserted c
onnectivities');
#20048=(
GEOMETRIC_REPRESENTATION_CONTEXT(3)
GLOBAL_UNCERTAINTY_ASSIGNED_CONTEXT((#19994))
GLOBAL_UNIT_ASSIGNED_CONTEXT((#20097,#20099,#20100))
REPRESENTATION_CONTEXT('','3D')
);
#20096=(
GEOMETRIC_REPRESENTATION_CONTEXT(3)
GLOBAL_UNCERTAINTY_ASSIGNED_CONTEXT((#20042))
GLOBAL_UNIT_ASSIGNED_CONTEXT((#20097,#20099,#20100))
REPRESENTATION_CONTEXT('','3D')
);
#20097=(
LENGTH_UNIT()
NAMED_UNIT(*)
SI_UNIT(.CENTI.,.METRE.)
);
#20099=(
NAMED_UNIT(*)
PLANE_ANGLE_UNIT()
SI_UNIT($,.RADIAN.)
);
#20100=(
NAMED_UNIT(*)
SI_UNIT($,.STERADIAN.)
SOLID_ANGLE_UNIT()
);
#20106=SHAPE_DEFINITION_REPRESENTATION(#20159,#20317);
#20159=PRODUCT_DEFINITION_SHAPE('',$,#20371);
#20317=SHAPE_REPRESENTATION('',(#11601),#20048);
#20365=PRODUCT_DEFINITION_CONTEXT('part definition',#20526,'design');
#20371=PRODUCT_DEFINITION('Fixed bearing block','Fixed bearing block',#20424,
#20365);
#20424=PRODUCT_DEFINITION_FORMATION('',$,#20533);
#20526=APPLICATION_CONTEXT(
'Core Data for Automotive Mechanical Design Process');
#20527=PRODUCT_CONTEXT('part definition',#20526,'mechanical');
#20533=PRODUCT('Fixed bearing block','Fixed bearing block',
'Fixed bearing block',(#20527));
#20644=COLOUR_RGB('Grey',0.48,0.52,0.57);
#20645=FILL_AREA_STYLE_COLOUR('',#20644);
#20646=FILL_AREA_STYLE('',(#20645));
#20647=SURFACE_STYLE_FILL_AREA(#20646);
#20648=SURFACE_SIDE_STYLE('',(#20647));
#20649=SURFACE_STYLE_USAGE(.BOTH.,#20648);
#20650=PRESENTATION_STYLE_ASSIGNMENT((#20649));
ENDSEC;
END-ISO-10303-21;
